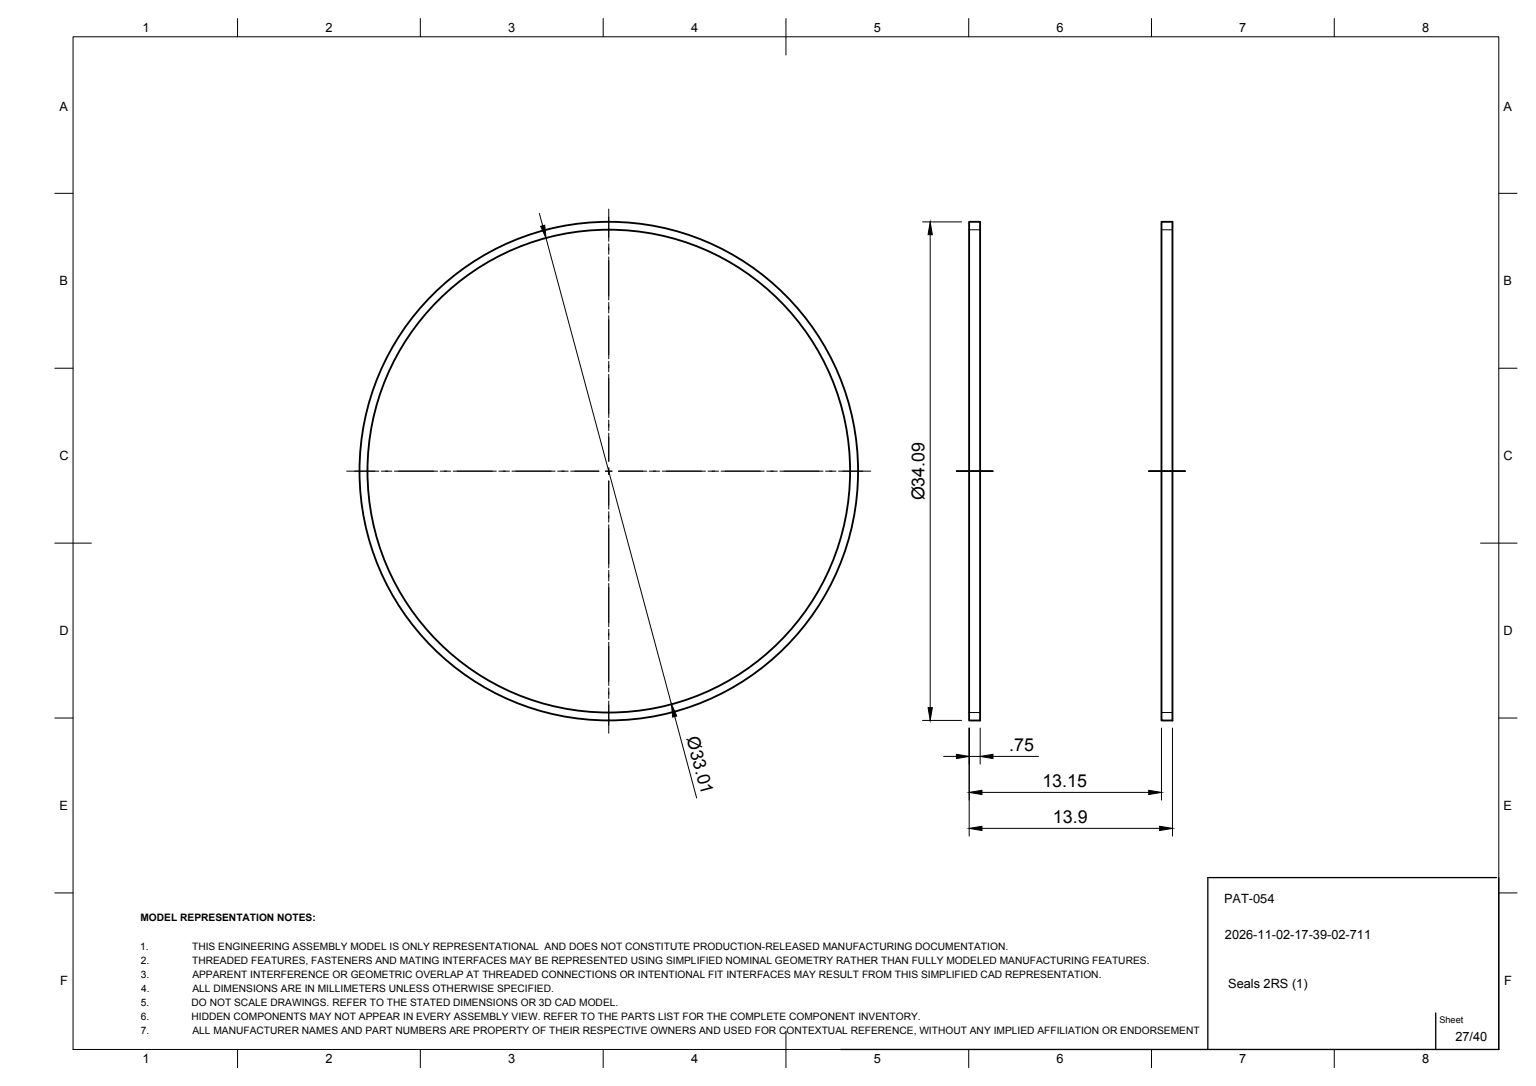
ISO-10303-21;
HEADER;
/* Generated by software containing ST-Developer
 * from STEP Tools, Inc. (www.steptools.com) 
 */

FILE_DESCRIPTION(
/* description */ ('PAT-054'),
/* implementation_level */ '2;1');

FILE_NAME(
/* name */ 'Seals 2RS (1).step',
/* time_stamp */ '2026-10-29T16:38:13-07:00',
/* author */ (''),
/* organization */ (''),
/* preprocessor_version */ 'ST-DEVELOPER v20.2',
/* originating_system */ 'Autodesk Translation Framework v15.17.0.0',
/* authorisation */ '');

FILE_SCHEMA (('AUTOMOTIVE_DESIGN { 1 0 10303 214 3 1 1 }'));
ENDSEC;

DATA;
#10=MECHANICAL_DESIGN_GEOMETRIC_PRESENTATION_REPRESENTATION('',(#931,#932),#33981);
#829=SHAPE_REPRESENTATION_RELATIONSHIP('SRR','None',#34204,#873);
#873=ADVANCED_BREP_SHAPE_REPRESENTATION('',(#990,#991),#33952);
#931=STYLED_ITEM('',(#34517),#990);
#932=STYLED_ITEM('',(#34517),#991);
#990=MANIFOLD_SOLID_BREP('Body1',#13042);
#991=MANIFOLD_SOLID_BREP('Body2',#13043);
#1142=FACE_BOUND('',#2673,.T.);
#1143=FACE_BOUND('',#2676,.T.);
#1144=FACE_BOUND('',#2679,.T.);
#1145=FACE_BOUND('',#2682,.T.);
#1340=PLANE('',#14112);
#1341=PLANE('',#14117);
#1342=PLANE('',#14120);
#1343=PLANE('',#14125);
#1819=FACE_OUTER_BOUND('',#2672,.T.);
#1820=FACE_OUTER_BOUND('',#2674,.T.);
#1821=FACE_OUTER_BOUND('',#2675,.T.);
#1822=FACE_OUTER_BOUND('',#2677,.T.);
#1823=FACE_OUTER_BOUND('',#2678,.T.);
#1824=FACE_OUTER_BOUND('',#2680,.T.);
#1825=FACE_OUTER_BOUND('',#2681,.T.);
#1826=FACE_OUTER_BOUND('',#2683,.T.);
#2672=EDGE_LOOP('',(#9613));
#2673=EDGE_LOOP('',(#9614));
#2674=EDGE_LOOP('',(#9615,#9616,#9617,#9618));
#2675=EDGE_LOOP('',(#9619));
#2676=EDGE_LOOP('',(#9620));
#2677=EDGE_LOOP('',(#9621,#9622,#9623,#9624));
#2678=EDGE_LOOP('',(#9625));
#2679=EDGE_LOOP('',(#9626));
#2680=EDGE_LOOP('',(#9627,#9628,#9629,#9630));
#2681=EDGE_LOOP('',(#9631));
#2682=EDGE_LOOP('',(#9632));
#2683=EDGE_LOOP('',(#9633,#9634,#9635,#9636));
#3486=LINE('',#20352,#4420);
#3487=LINE('',#20357,#4421);
#3488=LINE('',#20366,#4422);
#3489=LINE('',#20371,#4423);
#4420=VECTOR('',#16255,1.70469);
#4421=VECTOR('',#16262,1.65031);
#4422=VECTOR('',#16273,1.70469);
#4423=VECTOR('',#16280,1.65031);
#5386=CIRCLE('',#14113,1.70469);
#5387=CIRCLE('',#14114,1.65031);
#5388=CIRCLE('',#14116,1.70469);
#5389=CIRCLE('',#14118,1.65031);
#5390=CIRCLE('',#14121,1.70469);
#5391=CIRCLE('',#14122,1.65031);
#5392=CIRCLE('',#14124,1.70469);
#5393=CIRCLE('',#14126,1.65031);
#5962=VERTEX_POINT('',#20345);
#5963=VERTEX_POINT('',#20347);
#5964=VERTEX_POINT('',#20350);
#5965=VERTEX_POINT('',#20354);
#5966=VERTEX_POINT('',#20359);
#5967=VERTEX_POINT('',#20361);
#5968=VERTEX_POINT('',#20364);
#5969=VERTEX_POINT('',#20368);
#7306=EDGE_CURVE('',#5962,#5962,#5386,.T.);
#7307=EDGE_CURVE('',#5963,#5963,#5387,.T.);
#7308=EDGE_CURVE('',#5964,#5964,#5388,.T.);
#7309=EDGE_CURVE('',#5964,#5962,#3486,.T.);
#7310=EDGE_CURVE('',#5965,#5965,#5389,.T.);
#7311=EDGE_CURVE('',#5965,#5963,#3487,.T.);
#7312=EDGE_CURVE('',#5966,#5966,#5390,.T.);
#7313=EDGE_CURVE('',#5967,#5967,#5391,.T.);
#7314=EDGE_CURVE('',#5968,#5968,#5392,.T.);
#7315=EDGE_CURVE('',#5968,#5966,#3488,.T.);
#7316=EDGE_CURVE('',#5969,#5969,#5393,.T.);
#7317=EDGE_CURVE('',#5969,#5967,#3489,.T.);
#9613=ORIENTED_EDGE('',*,*,#7306,.F.);
#9614=ORIENTED_EDGE('',*,*,#7307,.T.);
#9615=ORIENTED_EDGE('',*,*,#7308,.F.);
#9616=ORIENTED_EDGE('',*,*,#7309,.T.);
#9617=ORIENTED_EDGE('',*,*,#7306,.T.);
#9618=ORIENTED_EDGE('',*,*,#7309,.F.);
#9619=ORIENTED_EDGE('',*,*,#7308,.T.);
#9620=ORIENTED_EDGE('',*,*,#7310,.F.);
#9621=ORIENTED_EDGE('',*,*,#7310,.T.);
#9622=ORIENTED_EDGE('',*,*,#7311,.T.);
#9623=ORIENTED_EDGE('',*,*,#7307,.F.);
#9624=ORIENTED_EDGE('',*,*,#7311,.F.);
#9625=ORIENTED_EDGE('',*,*,#7312,.F.);
#9626=ORIENTED_EDGE('',*,*,#7313,.T.);
#9627=ORIENTED_EDGE('',*,*,#7314,.F.);
#9628=ORIENTED_EDGE('',*,*,#7315,.T.);
#9629=ORIENTED_EDGE('',*,*,#7312,.T.);
#9630=ORIENTED_EDGE('',*,*,#7315,.F.);
#9631=ORIENTED_EDGE('',*,*,#7314,.T.);
#9632=ORIENTED_EDGE('',*,*,#7316,.F.);
#9633=ORIENTED_EDGE('',*,*,#7316,.T.);
#9634=ORIENTED_EDGE('',*,*,#7317,.T.);
#9635=ORIENTED_EDGE('',*,*,#7313,.F.);
#9636=ORIENTED_EDGE('',*,*,#7317,.F.);
#12069=CYLINDRICAL_SURFACE('',#14115,1.70469);
#12070=CYLINDRICAL_SURFACE('',#14119,1.65031);
#12071=CYLINDRICAL_SURFACE('',#14123,1.70469);
#12072=CYLINDRICAL_SURFACE('',#14127,1.65031);
#12531=ADVANCED_FACE('',(#1819,#1142),#1340,.T.);
#12532=ADVANCED_FACE('',(#1820),#12069,.T.);
#12533=ADVANCED_FACE('',(#1821,#1143),#1341,.T.);
#12534=ADVANCED_FACE('',(#1822),#12070,.F.);
#12535=ADVANCED_FACE('',(#1823,#1144),#1342,.T.);
#12536=ADVANCED_FACE('',(#1824),#12071,.T.);
#12537=ADVANCED_FACE('',(#1825,#1145),#1343,.T.);
#12538=ADVANCED_FACE('',(#1826),#12072,.F.);
#13042=CLOSED_SHELL('',(#12531,#12532,#12533,#12534));
#13043=CLOSED_SHELL('',(#12535,#12536,#12537,#12538));
#14111=AXIS2_PLACEMENT_3D('',#20343,#16243,#16244);
#14112=AXIS2_PLACEMENT_3D('',#20344,#16245,#16246);
#14113=AXIS2_PLACEMENT_3D('',#20346,#16247,#16248);
#14114=AXIS2_PLACEMENT_3D('',#20348,#16249,#16250);
#14115=AXIS2_PLACEMENT_3D('',#20349,#16251,#16252);
#14116=AXIS2_PLACEMENT_3D('',#20351,#16253,#16254);
#14117=AXIS2_PLACEMENT_3D('',#20353,#16256,#16257);
#14118=AXIS2_PLACEMENT_3D('',#20355,#16258,#16259);
#14119=AXIS2_PLACEMENT_3D('',#20356,#16260,#16261);
#14120=AXIS2_PLACEMENT_3D('',#20358,#16263,#16264);
#14121=AXIS2_PLACEMENT_3D('',#20360,#16265,#16266);
#14122=AXIS2_PLACEMENT_3D('',#20362,#16267,#16268);
#14123=AXIS2_PLACEMENT_3D('',#20363,#16269,#16270);
#14124=AXIS2_PLACEMENT_3D('',#20365,#16271,#16272);
#14125=AXIS2_PLACEMENT_3D('',#20367,#16274,#16275);
#14126=AXIS2_PLACEMENT_3D('',#20369,#16276,#16277);
#14127=AXIS2_PLACEMENT_3D('',#20370,#16278,#16279);
#16243=DIRECTION('axis',(0.,0.,1.));
#16244=DIRECTION('refdir',(1.,0.,0.));
#16245=DIRECTION('center_axis',(0.,1.,0.));
#16246=DIRECTION('ref_axis',(0.,0.,1.));
#16247=DIRECTION('center_axis',(0.,-1.,0.));
#16248=DIRECTION('ref_axis',(1.,0.,0.));
#16249=DIRECTION('center_axis',(0.,-1.,0.));
#16250=DIRECTION('ref_axis',(1.,0.,0.));
#16251=DIRECTION('center_axis',(0.,-1.,0.));
#16252=DIRECTION('ref_axis',(1.,0.,0.));
#16253=DIRECTION('center_axis',(0.,-1.,0.));
#16254=DIRECTION('ref_axis',(1.,0.,0.));
#16255=DIRECTION('',(0.,1.,0.));
#16256=DIRECTION('center_axis',(0.,-1.,0.));
#16257=DIRECTION('ref_axis',(0.,0.,-1.));
#16258=DIRECTION('center_axis',(0.,-1.,0.));
#16259=DIRECTION('ref_axis',(1.,0.,0.));
#16260=DIRECTION('center_axis',(0.,-1.,0.));
#16261=DIRECTION('ref_axis',(1.,0.,0.));
#16262=DIRECTION('',(0.,1.,0.));
#16263=DIRECTION('center_axis',(0.,1.,0.));
#16264=DIRECTION('ref_axis',(0.,0.,1.));
#16265=DIRECTION('center_axis',(0.,-1.,0.));
#16266=DIRECTION('ref_axis',(1.,0.,0.));
#16267=DIRECTION('center_axis',(0.,-1.,0.));
#16268=DIRECTION('ref_axis',(1.,0.,0.));
#16269=DIRECTION('center_axis',(0.,-1.,0.));
#16270=DIRECTION('ref_axis',(1.,0.,0.));
#16271=DIRECTION('center_axis',(0.,-1.,0.));
#16272=DIRECTION('ref_axis',(1.,0.,0.));
#16273=DIRECTION('',(0.,1.,0.));
#16274=DIRECTION('center_axis',(0.,-1.,0.));
#16275=DIRECTION('ref_axis',(0.,0.,-1.));
#16276=DIRECTION('center_axis',(0.,-1.,0.));
#16277=DIRECTION('ref_axis',(1.,0.,0.));
#16278=DIRECTION('center_axis',(0.,-1.,0.));
#16279=DIRECTION('ref_axis',(1.,0.,0.));
#16280=DIRECTION('',(0.,1.,0.));
#20343=CARTESIAN_POINT('',(0.,0.,0.));
#20344=CARTESIAN_POINT('Origin',(1.70469,0.695,0.));
#20345=CARTESIAN_POINT('',(-1.70469,0.695,-2.0876431520385E-16));
#20346=CARTESIAN_POINT('Origin',(0.,0.695,0.));
#20347=CARTESIAN_POINT('',(-1.65031,0.695,-2.02104685910087E-16));
#20348=CARTESIAN_POINT('Origin',(0.,0.695,0.));
#20349=CARTESIAN_POINT('Origin',(0.,0.6575,0.));
#20350=CARTESIAN_POINT('',(-1.70469,0.62,-2.0876431520385E-16));
#20351=CARTESIAN_POINT('Origin',(0.,0.62,0.));
#20352=CARTESIAN_POINT('',(-1.70469,0.6575,-2.0876431520385E-16));
#20353=CARTESIAN_POINT('Origin',(1.65031,0.62,0.));
#20354=CARTESIAN_POINT('',(-1.65031,0.62,-2.02104685910087E-16));
#20355=CARTESIAN_POINT('Origin',(0.,0.62,0.));
#20356=CARTESIAN_POINT('Origin',(0.,0.6575,0.));
#20357=CARTESIAN_POINT('',(-1.65031,0.6575,-2.02104685910087E-16));
#20358=CARTESIAN_POINT('Origin',(1.70469,-0.62,0.));
#20359=CARTESIAN_POINT('',(-1.70469,-0.62,-2.0876431520385E-16));
#20360=CARTESIAN_POINT('Origin',(0.,-0.62,0.));
#20361=CARTESIAN_POINT('',(-1.65031,-0.62,-2.02104685910087E-16));
#20362=CARTESIAN_POINT('Origin',(0.,-0.62,0.));
#20363=CARTESIAN_POINT('Origin',(0.,-0.6575,0.));
#20364=CARTESIAN_POINT('',(-1.70469,-0.695,-2.0876431520385E-16));
#20365=CARTESIAN_POINT('Origin',(0.,-0.695,0.));
#20366=CARTESIAN_POINT('',(-1.70469,-0.6575,-2.0876431520385E-16));
#20367=CARTESIAN_POINT('Origin',(1.65031,-0.695,0.));
#20368=CARTESIAN_POINT('',(-1.65031,-0.695,-2.02104685910087E-16));
#20369=CARTESIAN_POINT('Origin',(0.,-0.695,0.));
#20370=CARTESIAN_POINT('Origin',(0.,-0.6575,0.));
#20371=CARTESIAN_POINT('',(-1.65031,-0.6575,-2.02104685910087E-16));
#33900=UNCERTAINTY_MEASURE_WITH_UNIT(LENGTH_MEASURE(0.001),#33982,
'DISTANCE_ACCURACY_VALUE',
'Maximum model space distance between geometric entities at asserted c
onnectivities');
#33929=UNCERTAINTY_MEASURE_WITH_UNIT(LENGTH_MEASURE(0.001),#33982,
'DISTANCE_ACCURACY_VALUE',
'Maximum model space distance between geometric entities at asserted c
onnectivities');
#33952=(
GEOMETRIC_REPRESENTATION_CONTEXT(3)
GLOBAL_UNCERTAINTY_ASSIGNED_CONTEXT((#33900))
GLOBAL_UNIT_ASSIGNED_CONTEXT((#33982,#33984,#33985))
REPRESENTATION_CONTEXT('','3D')
);
#33981=(
GEOMETRIC_REPRESENTATION_CONTEXT(3)
GLOBAL_UNCERTAINTY_ASSIGNED_CONTEXT((#33929))
GLOBAL_UNIT_ASSIGNED_CONTEXT((#33982,#33984,#33985))
REPRESENTATION_CONTEXT('','3D')
);
#33982=(
LENGTH_UNIT()
NAMED_UNIT(*)
SI_UNIT(.CENTI.,.METRE.)
);
#33984=(
NAMED_UNIT(*)
PLANE_ANGLE_UNIT()
SI_UNIT($,.RADIAN.)
);
#33985=(
NAMED_UNIT(*)
SI_UNIT($,.STERADIAN.)
SOLID_ANGLE_UNIT()
);
#34008=SHAPE_DEFINITION_REPRESENTATION(#34064,#34204);
#34064=PRODUCT_DEFINITION_SHAPE('',$,#34256);
#34204=SHAPE_REPRESENTATION('',(#14111),#33952);
#34233=PRODUCT_DEFINITION_CONTEXT('part definition',#34388,'design');
#34256=PRODUCT_DEFINITION('Seals 2RS (1)','Seals 2RS (1)',#34307,#34233);
#34307=PRODUCT_DEFINITION_FORMATION('',$,#34412);
#34388=APPLICATION_CONTEXT(
'Core Data for Automotive Mechanical Design Process');
#34389=PRODUCT_CONTEXT('part definition',#34388,'mechanical');
#34412=PRODUCT('Seals 2RS (1)','Seals 2RS (1)','Seals 2RS (1)',(#34389));
#34511=COLOUR_RGB('Grey',0.48,0.52,0.57);
#34512=FILL_AREA_STYLE_COLOUR('',#34511);
#34513=FILL_AREA_STYLE('',(#34512));
#34514=SURFACE_STYLE_FILL_AREA(#34513);
#34515=SURFACE_SIDE_STYLE('',(#34514));
#34516=SURFACE_STYLE_USAGE(.BOTH.,#34515);
#34517=PRESENTATION_STYLE_ASSIGNMENT((#34516));
ENDSEC;
END-ISO-10303-21;
